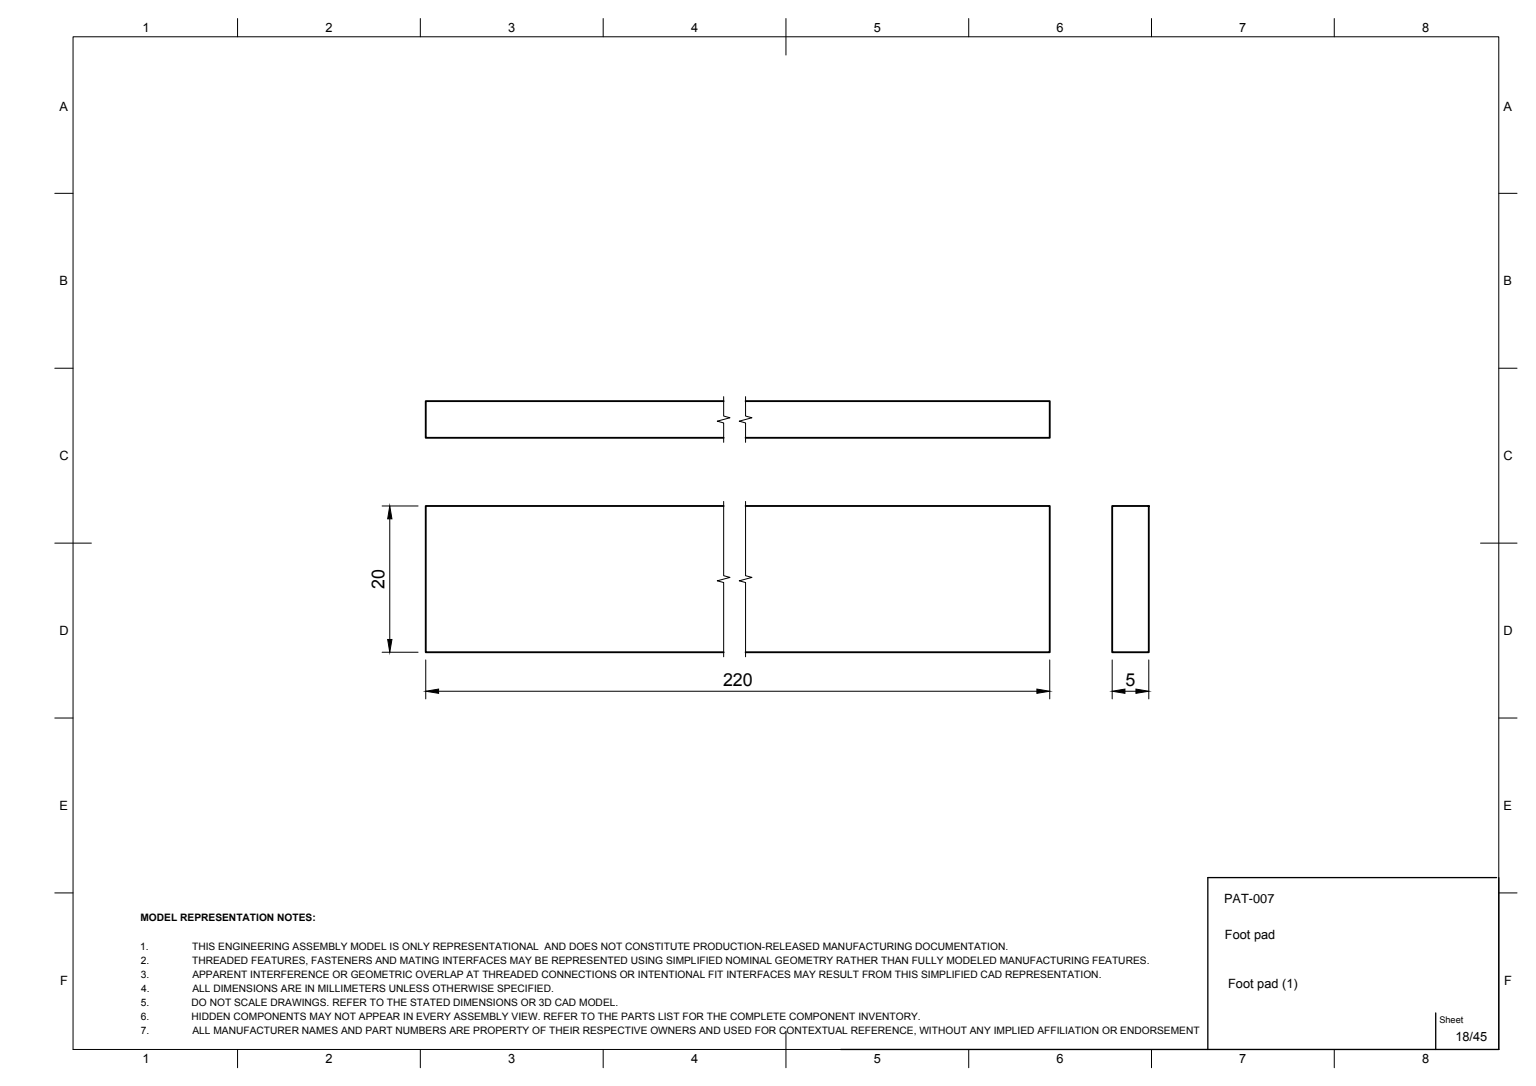
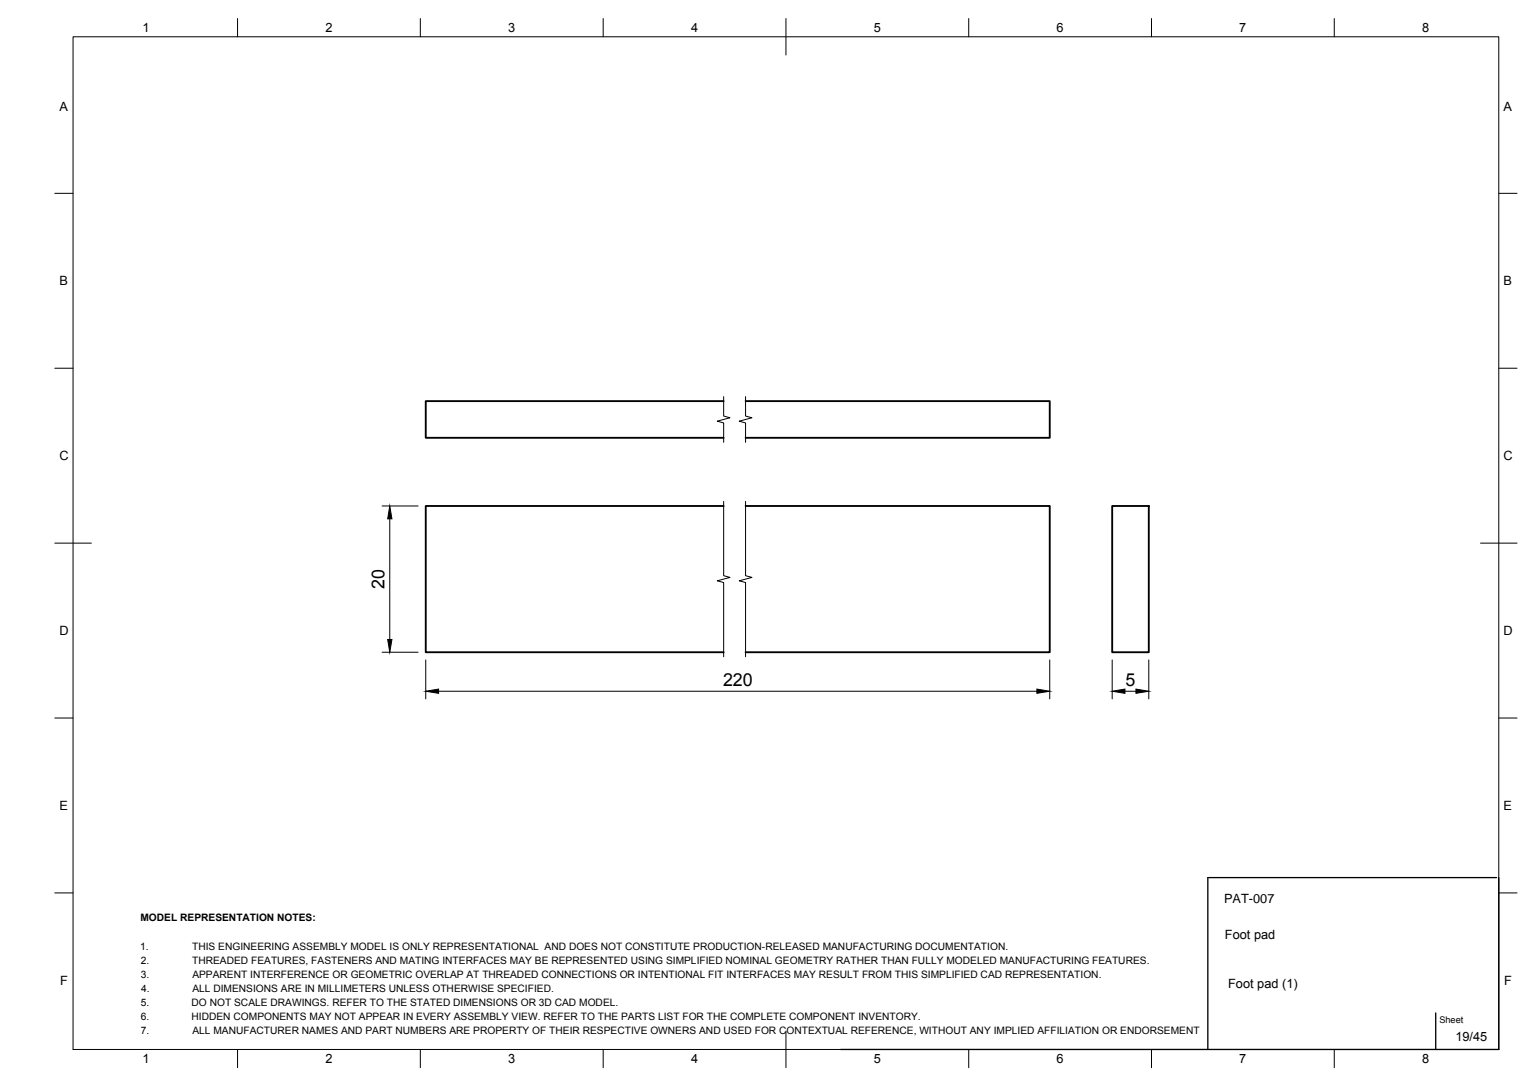
ISO-10303-21;
HEADER;
/* Generated by software containing ST-Developer
 * from STEP Tools, Inc. (www.steptools.com) 
 */

FILE_DESCRIPTION(
/* description */ ('Bearing friction torque test rig'),
/* implementation_level */ '2;1');

FILE_NAME(
/* name */ 'Foot pad (1).step',
/* time_stamp */ '2026-10-28T03:24:04-07:00',
/* author */ (''),
/* organization */ (''),
/* preprocessor_version */ 'ST-DEVELOPER v20.2',
/* originating_system */ 'Autodesk Translation Framework v15.17.0.0',
/* authorisation */ '');

FILE_SCHEMA (('AUTOMOTIVE_DESIGN { 1 0 10303 214 3 1 1 }'));
ENDSEC;

DATA;
#10=MECHANICAL_DESIGN_GEOMETRIC_PRESENTATION_REPRESENTATION('',(#553),#14822);
#475=SHAPE_REPRESENTATION_RELATIONSHIP('SRR','None',#15014,#514);
#514=ADVANCED_BREP_SHAPE_REPRESENTATION('',(#607),#14794);
#553=STYLED_ITEM('',(#15277),#607);
#607=MANIFOLD_SOLID_BREP('Body1',#7669);
#985=PLANE('',#8592);
#986=PLANE('',#8593);
#987=PLANE('',#8594);
#988=PLANE('',#8595);
#989=PLANE('',#8596);
#990=PLANE('',#8597);
#1314=FACE_OUTER_BOUND('',#1928,.T.);
#1315=FACE_OUTER_BOUND('',#1929,.T.);
#1316=FACE_OUTER_BOUND('',#1930,.T.);
#1317=FACE_OUTER_BOUND('',#1931,.T.);
#1318=FACE_OUTER_BOUND('',#1932,.T.);
#1319=FACE_OUTER_BOUND('',#1933,.T.);
#1928=EDGE_LOOP('',(#6120,#6121,#6122,#6123));
#1929=EDGE_LOOP('',(#6124,#6125,#6126,#6127));
#1930=EDGE_LOOP('',(#6128,#6129,#6130,#6131));
#1931=EDGE_LOOP('',(#6132,#6133,#6134,#6135));
#1932=EDGE_LOOP('',(#6136,#6137,#6138,#6139));
#1933=EDGE_LOOP('',(#6140,#6141,#6142,#6143));
#2487=LINE('',#12703,#2931);
#2488=LINE('',#12705,#2932);
#2489=LINE('',#12707,#2933);
#2490=LINE('',#12708,#2934);
#2491=LINE('',#12711,#2935);
#2492=LINE('',#12713,#2936);
#2493=LINE('',#12714,#2937);
#2494=LINE('',#12717,#2938);
#2495=LINE('',#12719,#2939);
#2496=LINE('',#12720,#2940);
#2497=LINE('',#12722,#2941);
#2498=LINE('',#12723,#2942);
#2931=VECTOR('',#10336,1.);
#2932=VECTOR('',#10337,1.);
#2933=VECTOR('',#10338,1.);
#2934=VECTOR('',#10339,1.);
#2935=VECTOR('',#10342,1.);
#2936=VECTOR('',#10343,1.);
#2937=VECTOR('',#10344,1.);
#2938=VECTOR('',#10347,1.);
#2939=VECTOR('',#10348,1.);
#2940=VECTOR('',#10349,1.);
#2941=VECTOR('',#10352,1.);
#2942=VECTOR('',#10353,1.);
#3877=VERTEX_POINT('',#12701);
#3878=VERTEX_POINT('',#12702);
#3879=VERTEX_POINT('',#12704);
#3880=VERTEX_POINT('',#12706);
#3881=VERTEX_POINT('',#12710);
#3882=VERTEX_POINT('',#12712);
#3883=VERTEX_POINT('',#12716);
#3884=VERTEX_POINT('',#12718);
#4686=EDGE_CURVE('',#3877,#3878,#2487,.T.);
#4687=EDGE_CURVE('',#3878,#3879,#2488,.T.);
#4688=EDGE_CURVE('',#3880,#3879,#2489,.T.);
#4689=EDGE_CURVE('',#3877,#3880,#2490,.T.);
#4690=EDGE_CURVE('',#3881,#3877,#2491,.T.);
#4691=EDGE_CURVE('',#3882,#3880,#2492,.T.);
#4692=EDGE_CURVE('',#3881,#3882,#2493,.T.);
#4693=EDGE_CURVE('',#3883,#3881,#2494,.T.);
#4694=EDGE_CURVE('',#3884,#3882,#2495,.T.);
#4695=EDGE_CURVE('',#3883,#3884,#2496,.T.);
#4696=EDGE_CURVE('',#3878,#3883,#2497,.T.);
#4697=EDGE_CURVE('',#3879,#3884,#2498,.T.);
#6120=ORIENTED_EDGE('',*,*,#4686,.T.);
#6121=ORIENTED_EDGE('',*,*,#4687,.T.);
#6122=ORIENTED_EDGE('',*,*,#4688,.F.);
#6123=ORIENTED_EDGE('',*,*,#4689,.F.);
#6124=ORIENTED_EDGE('',*,*,#4690,.T.);
#6125=ORIENTED_EDGE('',*,*,#4689,.T.);
#6126=ORIENTED_EDGE('',*,*,#4691,.F.);
#6127=ORIENTED_EDGE('',*,*,#4692,.F.);
#6128=ORIENTED_EDGE('',*,*,#4693,.T.);
#6129=ORIENTED_EDGE('',*,*,#4692,.T.);
#6130=ORIENTED_EDGE('',*,*,#4694,.F.);
#6131=ORIENTED_EDGE('',*,*,#4695,.F.);
#6132=ORIENTED_EDGE('',*,*,#4696,.T.);
#6133=ORIENTED_EDGE('',*,*,#4695,.T.);
#6134=ORIENTED_EDGE('',*,*,#4697,.F.);
#6135=ORIENTED_EDGE('',*,*,#4687,.F.);
#6136=ORIENTED_EDGE('',*,*,#4697,.T.);
#6137=ORIENTED_EDGE('',*,*,#4694,.T.);
#6138=ORIENTED_EDGE('',*,*,#4691,.T.);
#6139=ORIENTED_EDGE('',*,*,#4688,.T.);
#6140=ORIENTED_EDGE('',*,*,#4696,.F.);
#6141=ORIENTED_EDGE('',*,*,#4686,.F.);
#6142=ORIENTED_EDGE('',*,*,#4690,.F.);
#6143=ORIENTED_EDGE('',*,*,#4693,.F.);
#7425=ADVANCED_FACE('',(#1314),#985,.T.);
#7426=ADVANCED_FACE('',(#1315),#986,.T.);
#7427=ADVANCED_FACE('',(#1316),#987,.T.);
#7428=ADVANCED_FACE('',(#1317),#988,.T.);
#7429=ADVANCED_FACE('',(#1318),#989,.T.);
#7430=ADVANCED_FACE('',(#1319),#990,.F.);
#7669=CLOSED_SHELL('',(#7425,#7426,#7427,#7428,#7429,#7430));
#8591=AXIS2_PLACEMENT_3D('',#12699,#10332,#10333);
#8592=AXIS2_PLACEMENT_3D('',#12700,#10334,#10335);
#8593=AXIS2_PLACEMENT_3D('',#12709,#10340,#10341);
#8594=AXIS2_PLACEMENT_3D('',#12715,#10345,#10346);
#8595=AXIS2_PLACEMENT_3D('',#12721,#10350,#10351);
#8596=AXIS2_PLACEMENT_3D('',#12724,#10354,#10355);
#8597=AXIS2_PLACEMENT_3D('',#12725,#10356,#10357);
#10332=DIRECTION('axis',(0.,0.,1.));
#10333=DIRECTION('refdir',(1.,0.,0.));
#10334=DIRECTION('center_axis',(0.,1.,0.));
#10335=DIRECTION('ref_axis',(-1.,0.,0.));
#10336=DIRECTION('',(-1.,0.,0.));
#10337=DIRECTION('',(0.,0.,1.));
#10338=DIRECTION('',(-1.,0.,0.));
#10339=DIRECTION('',(0.,0.,1.));
#10340=DIRECTION('center_axis',(1.,0.,0.));
#10341=DIRECTION('ref_axis',(0.,1.,0.));
#10342=DIRECTION('',(0.,1.,0.));
#10343=DIRECTION('',(0.,1.,0.));
#10344=DIRECTION('',(0.,0.,1.));
#10345=DIRECTION('center_axis',(0.,-1.,0.));
#10346=DIRECTION('ref_axis',(1.,0.,0.));
#10347=DIRECTION('',(1.,0.,0.));
#10348=DIRECTION('',(1.,0.,0.));
#10349=DIRECTION('',(0.,0.,1.));
#10350=DIRECTION('center_axis',(-1.,0.,0.));
#10351=DIRECTION('ref_axis',(0.,-1.,0.));
#10352=DIRECTION('',(0.,-1.,0.));
#10353=DIRECTION('',(0.,-1.,0.));
#10354=DIRECTION('center_axis',(0.,0.,1.));
#10355=DIRECTION('ref_axis',(1.,0.,0.));
#10356=DIRECTION('center_axis',(0.,0.,1.));
#10357=DIRECTION('ref_axis',(1.,0.,0.));
#12699=CARTESIAN_POINT('',(0.,0.,0.));
#12700=CARTESIAN_POINT('Origin',(12.5,11.,-0.5));
#12701=CARTESIAN_POINT('',(12.5,11.,-0.5));
#12702=CARTESIAN_POINT('',(10.5,11.,-0.5));
#12703=CARTESIAN_POINT('',(12.5,11.,-0.5));
#12704=CARTESIAN_POINT('',(10.5,11.,0.));
#12705=CARTESIAN_POINT('',(10.5,11.,-0.5));
#12706=CARTESIAN_POINT('',(12.5,11.,0.));
#12707=CARTESIAN_POINT('',(12.5,11.,0.));
#12708=CARTESIAN_POINT('',(12.5,11.,-0.5));
#12709=CARTESIAN_POINT('Origin',(12.5,-11.,-0.5));
#12710=CARTESIAN_POINT('',(12.5,-11.,-0.5));
#12711=CARTESIAN_POINT('',(12.5,-11.,-0.5));
#12712=CARTESIAN_POINT('',(12.5,-11.,0.));
#12713=CARTESIAN_POINT('',(12.5,-11.,0.));
#12714=CARTESIAN_POINT('',(12.5,-11.,-0.5));
#12715=CARTESIAN_POINT('Origin',(10.5,-11.,-0.5));
#12716=CARTESIAN_POINT('',(10.5,-11.,-0.5));
#12717=CARTESIAN_POINT('',(10.5,-11.,-0.5));
#12718=CARTESIAN_POINT('',(10.5,-11.,0.));
#12719=CARTESIAN_POINT('',(10.5,-11.,0.));
#12720=CARTESIAN_POINT('',(10.5,-11.,-0.5));
#12721=CARTESIAN_POINT('Origin',(10.5,11.,-0.5));
#12722=CARTESIAN_POINT('',(10.5,11.,-0.5));
#12723=CARTESIAN_POINT('',(10.5,11.,0.));
#12724=CARTESIAN_POINT('Origin',(11.5,0.,0.));
#12725=CARTESIAN_POINT('Origin',(11.5,0.,-0.5));
#14749=UNCERTAINTY_MEASURE_WITH_UNIT(LENGTH_MEASURE(0.001),#14823,
'DISTANCE_ACCURACY_VALUE',
'Maximum model space distance between geometric entities at asserted c
onnectivities');
#14777=UNCERTAINTY_MEASURE_WITH_UNIT(LENGTH_MEASURE(0.001),#14823,
'DISTANCE_ACCURACY_VALUE',
'Maximum model space distance between geometric entities at asserted c
onnectivities');
#14794=(
GEOMETRIC_REPRESENTATION_CONTEXT(3)
GLOBAL_UNCERTAINTY_ASSIGNED_CONTEXT((#14749))
GLOBAL_UNIT_ASSIGNED_CONTEXT((#14823,#14825,#14826))
REPRESENTATION_CONTEXT('','3D')
);
#14822=(
GEOMETRIC_REPRESENTATION_CONTEXT(3)
GLOBAL_UNCERTAINTY_ASSIGNED_CONTEXT((#14777))
GLOBAL_UNIT_ASSIGNED_CONTEXT((#14823,#14825,#14826))
REPRESENTATION_CONTEXT('','3D')
);
#14823=(
LENGTH_UNIT()
NAMED_UNIT(*)
SI_UNIT(.CENTI.,.METRE.)
);
#14825=(
NAMED_UNIT(*)
PLANE_ANGLE_UNIT()
SI_UNIT($,.RADIAN.)
);
#14826=(
NAMED_UNIT(*)
SI_UNIT($,.STERADIAN.)
SOLID_ANGLE_UNIT()
);
#14843=SHAPE_DEFINITION_REPRESENTATION(#14887,#15014);
#14887=PRODUCT_DEFINITION_SHAPE('',$,#15059);
#15014=SHAPE_REPRESENTATION('',(#8591),#14794);
#15042=PRODUCT_DEFINITION_CONTEXT('part definition',#15176,'design');
#15059=PRODUCT_DEFINITION('Foot pad (1)','Foot pad (1)',#15103,#15042);
#15103=PRODUCT_DEFINITION_FORMATION('',$,#15194);
#15176=APPLICATION_CONTEXT(
'Core Data for Automotive Mechanical Design Process');
#15177=PRODUCT_CONTEXT('part definition',#15176,'mechanical');
#15194=PRODUCT('Foot pad (1)','Foot pad (1)','Foot pad (1)',(#15177));
#15271=COLOUR_RGB('Sky Blue',0.24,0.69,0.87);
#15272=FILL_AREA_STYLE_COLOUR('',#15271);
#15273=FILL_AREA_STYLE('',(#15272));
#15274=SURFACE_STYLE_FILL_AREA(#15273);
#15275=SURFACE_SIDE_STYLE('',(#15274));
#15276=SURFACE_STYLE_USAGE(.BOTH.,#15275);
#15277=PRESENTATION_STYLE_ASSIGNMENT((#15276));
ENDSEC;
END-ISO-10303-21;
